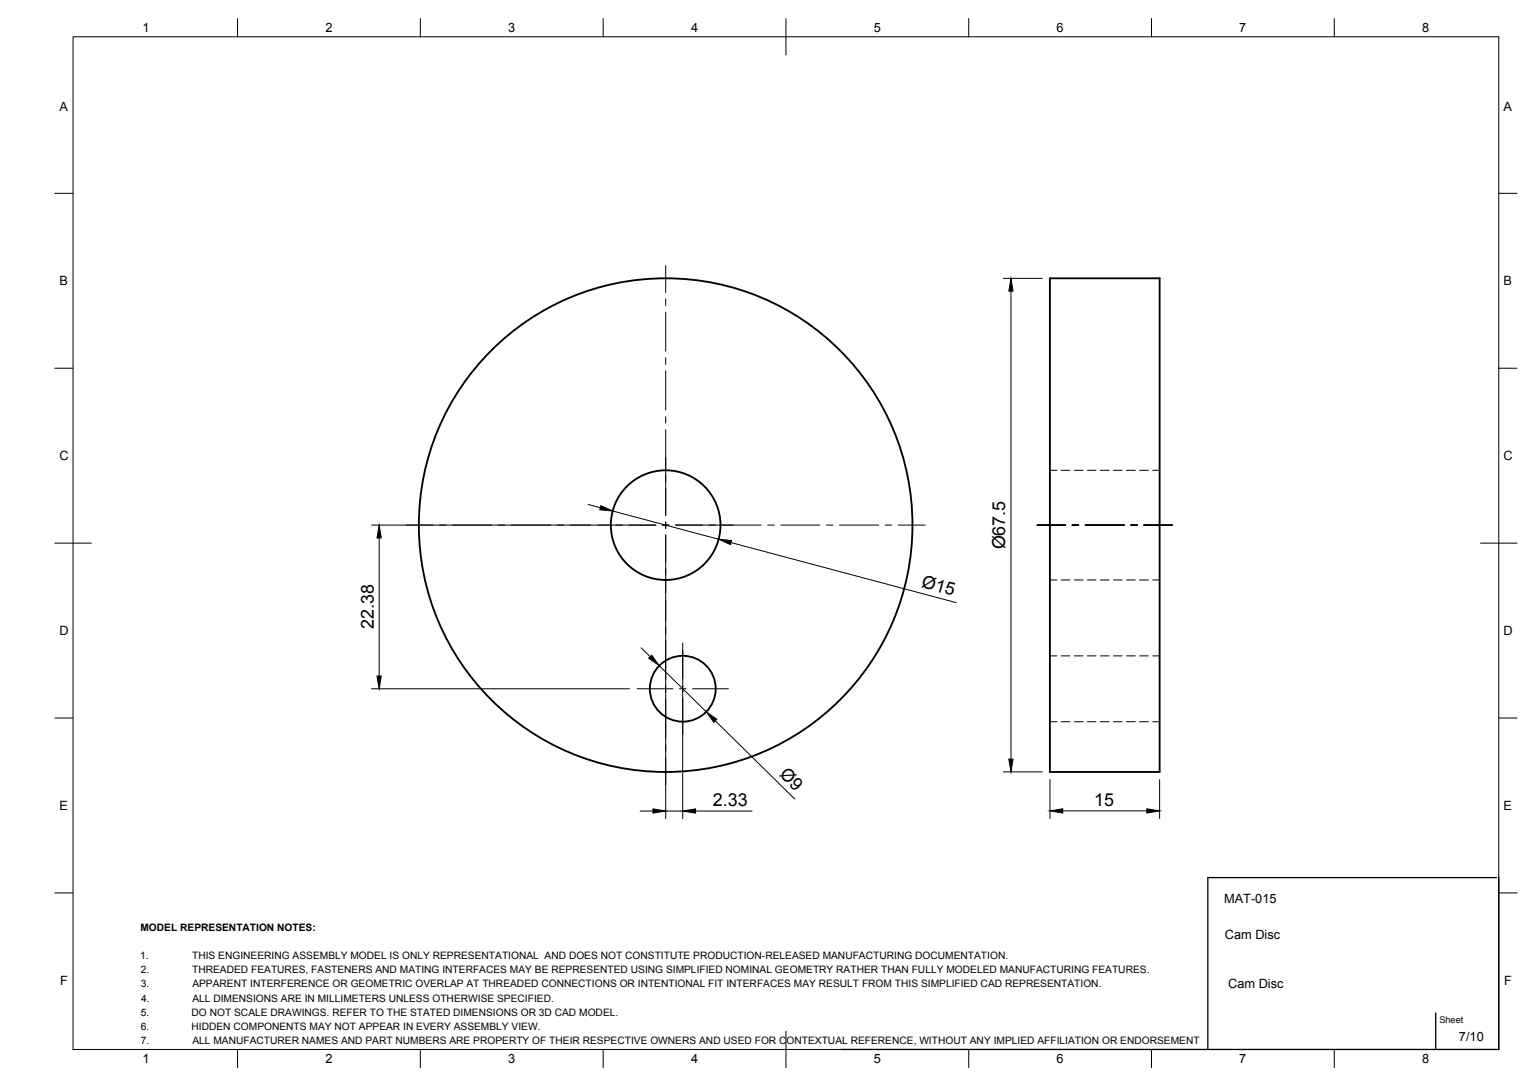
ISO-10303-21;
HEADER;
/* Generated by software containing ST-Developer
 * from STEP Tools, Inc. (www.steptools.com) 
 */

FILE_DESCRIPTION(
/* description */ ('STEP AP214'),
/* implementation_level */ '2;1');

FILE_NAME(
/* name */ 'Cam Disc.step',
/* time_stamp */ '2026-11-14T06:03:18-08:00',
/* author */ (''),
/* organization */ (''),
/* preprocessor_version */ 'ST-DEVELOPER v20.2',
/* originating_system */ 'Autodesk Translation Framework v15.17.0.0',
/* authorisation */ '');

FILE_SCHEMA (('AUTOMOTIVE_DESIGN { 1 0 10303 214 3 1 1 }'));
ENDSEC;

DATA;
#10=MECHANICAL_DESIGN_GEOMETRIC_PRESENTATION_REPRESENTATION('',(#75),#3206);
#59=SHAPE_REPRESENTATION_RELATIONSHIP('SRR','None',#3242,#67);
#67=ADVANCED_BREP_SHAPE_REPRESENTATION('',(#83),#3201);
#75=STYLED_ITEM('',(#3289),#83);
#83=MANIFOLD_SOLID_BREP('Body1',#1782);
#109=PLANE('',#1959);
#110=PLANE('',#1960);
#160=FACE_BOUND('',#666,.T.);
#161=FACE_BOUND('',#667,.T.);
#162=FACE_BOUND('',#669,.T.);
#163=FACE_BOUND('',#670,.T.);
#224=LINE('',#2852,#369);
#225=LINE('',#2858,#370);
#226=LINE('',#2864,#371);
#369=VECTOR('',#2263,4.50000000000001);
#370=VECTOR('',#2270,7.50000000000002);
#371=VECTOR('',#2277,33.7500000000001);
#489=CYLINDRICAL_SURFACE('',#1950,4.50000000000001);
#490=CYLINDRICAL_SURFACE('',#1953,7.50000000000002);
#491=CYLINDRICAL_SURFACE('',#1956,33.7500000000001);
#549=FACE_OUTER_BOUND('',#662,.T.);
#550=FACE_OUTER_BOUND('',#663,.T.);
#551=FACE_OUTER_BOUND('',#664,.T.);
#552=FACE_OUTER_BOUND('',#665,.T.);
#553=FACE_OUTER_BOUND('',#668,.T.);
#662=EDGE_LOOP('',(#1361,#1362,#1363,#1364));
#663=EDGE_LOOP('',(#1365,#1366,#1367,#1368));
#664=EDGE_LOOP('',(#1369,#1370,#1371,#1372));
#665=EDGE_LOOP('',(#1373));
#666=EDGE_LOOP('',(#1374));
#667=EDGE_LOOP('',(#1375));
#668=EDGE_LOOP('',(#1376));
#669=EDGE_LOOP('',(#1377));
#670=EDGE_LOOP('',(#1378));
#785=CIRCLE('',#1951,4.50000000000001);
#786=CIRCLE('',#1952,4.50000000000001);
#787=CIRCLE('',#1954,7.50000000000002);
#788=CIRCLE('',#1955,7.50000000000002);
#789=CIRCLE('',#1957,33.7500000000001);
#790=CIRCLE('',#1958,33.7500000000001);
#882=VERTEX_POINT('',#2849);
#883=VERTEX_POINT('',#2851);
#884=VERTEX_POINT('',#2855);
#885=VERTEX_POINT('',#2857);
#886=VERTEX_POINT('',#2861);
#887=VERTEX_POINT('',#2863);
#1059=EDGE_CURVE('',#882,#882,#785,.T.);
#1060=EDGE_CURVE('',#882,#883,#224,.T.);
#1061=EDGE_CURVE('',#883,#883,#786,.T.);
#1062=EDGE_CURVE('',#884,#884,#787,.T.);
#1063=EDGE_CURVE('',#884,#885,#225,.T.);
#1064=EDGE_CURVE('',#885,#885,#788,.T.);
#1065=EDGE_CURVE('',#886,#886,#789,.T.);
#1066=EDGE_CURVE('',#886,#887,#226,.T.);
#1067=EDGE_CURVE('',#887,#887,#790,.T.);
#1361=ORIENTED_EDGE('',*,*,#1059,.T.);
#1362=ORIENTED_EDGE('',*,*,#1060,.T.);
#1363=ORIENTED_EDGE('',*,*,#1061,.F.);
#1364=ORIENTED_EDGE('',*,*,#1060,.F.);
#1365=ORIENTED_EDGE('',*,*,#1062,.T.);
#1366=ORIENTED_EDGE('',*,*,#1063,.T.);
#1367=ORIENTED_EDGE('',*,*,#1064,.F.);
#1368=ORIENTED_EDGE('',*,*,#1063,.F.);
#1369=ORIENTED_EDGE('',*,*,#1065,.T.);
#1370=ORIENTED_EDGE('',*,*,#1066,.T.);
#1371=ORIENTED_EDGE('',*,*,#1067,.F.);
#1372=ORIENTED_EDGE('',*,*,#1066,.F.);
#1373=ORIENTED_EDGE('',*,*,#1067,.T.);
#1374=ORIENTED_EDGE('',*,*,#1059,.F.);
#1375=ORIENTED_EDGE('',*,*,#1062,.F.);
#1376=ORIENTED_EDGE('',*,*,#1065,.F.);
#1377=ORIENTED_EDGE('',*,*,#1061,.T.);
#1378=ORIENTED_EDGE('',*,*,#1064,.T.);
#1716=ADVANCED_FACE('',(#549),#489,.F.);
#1717=ADVANCED_FACE('',(#550),#490,.F.);
#1718=ADVANCED_FACE('',(#551),#491,.T.);
#1719=ADVANCED_FACE('',(#552,#160,#161),#109,.T.);
#1720=ADVANCED_FACE('',(#553,#162,#163),#110,.F.);
#1782=CLOSED_SHELL('',(#1716,#1717,#1718,#1719,#1720));
#1949=AXIS2_PLACEMENT_3D('',#2847,#2257,#2258);
#1950=AXIS2_PLACEMENT_3D('',#2848,#2259,#2260);
#1951=AXIS2_PLACEMENT_3D('',#2850,#2261,#2262);
#1952=AXIS2_PLACEMENT_3D('',#2853,#2264,#2265);
#1953=AXIS2_PLACEMENT_3D('',#2854,#2266,#2267);
#1954=AXIS2_PLACEMENT_3D('',#2856,#2268,#2269);
#1955=AXIS2_PLACEMENT_3D('',#2859,#2271,#2272);
#1956=AXIS2_PLACEMENT_3D('',#2860,#2273,#2274);
#1957=AXIS2_PLACEMENT_3D('',#2862,#2275,#2276);
#1958=AXIS2_PLACEMENT_3D('',#2865,#2278,#2279);
#1959=AXIS2_PLACEMENT_3D('',#2866,#2280,#2281);
#1960=AXIS2_PLACEMENT_3D('',#2867,#2282,#2283);
#2257=DIRECTION('axis',(0.,0.,1.));
#2258=DIRECTION('refdir',(1.,0.,0.));
#2259=DIRECTION('center_axis',(-1.87200390594439E-31,-2.8065614114583E-31,
-1.));
#2260=DIRECTION('ref_axis',(-1.,5.25389392452275E-62,1.87200390594439E-31));
#2261=DIRECTION('center_axis',(1.87200390594439E-31,2.8065614114583E-31,
1.));
#2262=DIRECTION('ref_axis',(1.,-5.25389392452275E-62,-1.87200390594439E-31));
#2263=DIRECTION('',(-1.87200390594439E-31,-2.8065614114583E-31,-1.));
#2264=DIRECTION('center_axis',(1.87200390594439E-31,2.8065614114583E-31,
1.));
#2265=DIRECTION('ref_axis',(1.,-5.25389392452275E-62,-1.87200390594439E-31));
#2266=DIRECTION('center_axis',(-1.87200390594439E-31,-2.8065614114583E-31,
-1.));
#2267=DIRECTION('ref_axis',(-1.,-2.89120579329467E-17,1.87200390594439E-31));
#2268=DIRECTION('center_axis',(1.87200390594439E-31,2.8065614114583E-31,
1.));
#2269=DIRECTION('ref_axis',(1.,2.89120579329467E-17,-1.87200390594439E-31));
#2270=DIRECTION('',(-1.87200390594439E-31,-2.8065614114583E-31,-1.));
#2271=DIRECTION('center_axis',(1.87200390594439E-31,2.8065614114583E-31,
1.));
#2272=DIRECTION('ref_axis',(1.,2.89120579329467E-17,-1.87200390594439E-31));
#2273=DIRECTION('center_axis',(-1.87200390594439E-31,-2.8065614114583E-31,
-1.));
#2274=DIRECTION('ref_axis',(-1.,-2.81089452125871E-17,1.87200390594439E-31));
#2275=DIRECTION('center_axis',(1.87200390594439E-31,2.8065614114583E-31,
1.));
#2276=DIRECTION('ref_axis',(1.,2.81089452125871E-17,-1.87200390594439E-31));
#2277=DIRECTION('',(1.87200390594439E-31,2.8065614114583E-31,1.));
#2278=DIRECTION('center_axis',(1.87200390594439E-31,2.8065614114583E-31,
1.));
#2279=DIRECTION('ref_axis',(1.,2.81089452125871E-17,-1.87200390594439E-31));
#2280=DIRECTION('center_axis',(-1.85852239633368E-31,2.8065614114583E-31,
1.));
#2281=DIRECTION('ref_axis',(1.,2.77555756156288E-17,1.85852239633368E-31));
#2282=DIRECTION('center_axis',(-1.85852239633368E-31,2.8065614114583E-31,
1.));
#2283=DIRECTION('ref_axis',(1.,2.77555756156288E-17,1.85852239633368E-31));
#2847=CARTESIAN_POINT('',(0.,0.,0.));
#2848=CARTESIAN_POINT('Origin',(-6.93889390390723E-15,22.6429327686607,
12.5));
#2849=CARTESIAN_POINT('',(4.50000000000001,22.6429327686607,12.5));
#2850=CARTESIAN_POINT('Origin',(-6.93889390390723E-15,22.6429327686607,
12.5));
#2851=CARTESIAN_POINT('',(4.50000000000001,22.6429327686607,-2.5));
#2852=CARTESIAN_POINT('',(4.50000000000001,22.6429327686607,12.5));
#2853=CARTESIAN_POINT('Origin',(-6.93889390390723E-15,22.6429327686607,
-2.5));
#2854=CARTESIAN_POINT('Origin',(0.,0.142932768660666,12.5));
#2855=CARTESIAN_POINT('',(7.50000000000002,0.142932768660665,12.5));
#2856=CARTESIAN_POINT('Origin',(0.,0.142932768660666,12.5));
#2857=CARTESIAN_POINT('',(7.50000000000002,0.142932768660665,-2.5));
#2858=CARTESIAN_POINT('',(7.50000000000002,0.142932768660665,12.5));
#2859=CARTESIAN_POINT('Origin',(0.,0.142932768660666,-2.5));
#2860=CARTESIAN_POINT('Origin',(0.,0.142932768660666,12.5));
#2861=CARTESIAN_POINT('',(33.7500000000001,0.142932768660662,-2.5));
#2862=CARTESIAN_POINT('Origin',(0.,0.142932768660666,-2.5));
#2863=CARTESIAN_POINT('',(33.7500000000001,0.142932768660662,12.5));
#2864=CARTESIAN_POINT('',(33.7500000000001,0.142932768660662,12.5));
#2865=CARTESIAN_POINT('Origin',(0.,0.142932768660666,12.5));
#2866=CARTESIAN_POINT('Origin',(0.,0.142932768660666,12.5));
#2867=CARTESIAN_POINT('Origin',(0.,0.142932768660666,-2.5));
#3191=UNCERTAINTY_MEASURE_WITH_UNIT(LENGTH_MEASURE(0.01),#3207,
'DISTANCE_ACCURACY_VALUE',
'Maximum model space distance between geometric entities at asserted c
onnectivities');
#3196=UNCERTAINTY_MEASURE_WITH_UNIT(LENGTH_MEASURE(0.01),#3207,
'DISTANCE_ACCURACY_VALUE',
'Maximum model space distance between geometric entities at asserted c
onnectivities');
#3201=(
GEOMETRIC_REPRESENTATION_CONTEXT(3)
GLOBAL_UNCERTAINTY_ASSIGNED_CONTEXT((#3191))
GLOBAL_UNIT_ASSIGNED_CONTEXT((#3207,#3209,#3210))
REPRESENTATION_CONTEXT('','3D')
);
#3206=(
GEOMETRIC_REPRESENTATION_CONTEXT(3)
GLOBAL_UNCERTAINTY_ASSIGNED_CONTEXT((#3196))
GLOBAL_UNIT_ASSIGNED_CONTEXT((#3207,#3209,#3210))
REPRESENTATION_CONTEXT('','3D')
);
#3207=(
LENGTH_UNIT()
NAMED_UNIT(*)
SI_UNIT(.MILLI.,.METRE.)
);
#3209=(
NAMED_UNIT(*)
PLANE_ANGLE_UNIT()
SI_UNIT($,.RADIAN.)
);
#3210=(
NAMED_UNIT(*)
SI_UNIT($,.STERADIAN.)
SOLID_ANGLE_UNIT()
);
#3215=SHAPE_DEFINITION_REPRESENTATION(#3224,#3242);
#3224=PRODUCT_DEFINITION_SHAPE('',$,#3252);
#3242=SHAPE_REPRESENTATION('',(#1949),#3201);
#3247=PRODUCT_DEFINITION_CONTEXT('part definition',#3276,'design');
#3252=PRODUCT_DEFINITION('Cam Disc','Cam Disc',#3261,#3247);
#3261=PRODUCT_DEFINITION_FORMATION('',$,#3282);
#3276=APPLICATION_CONTEXT(
'Core Data for Automotive Mechanical Design Process');
#3277=PRODUCT_CONTEXT('part definition',#3276,'mechanical');
#3282=PRODUCT('Cam Disc','Cam Disc',$,(#3277));
#3289=PRESENTATION_STYLE_ASSIGNMENT((#3293));
#3293=SURFACE_STYLE_USAGE(.BOTH.,#3297);
#3297=SURFACE_SIDE_STYLE('',(#3301));
#3301=SURFACE_STYLE_FILL_AREA(#3305);
#3305=FILL_AREA_STYLE('Opaque(97,158,199)',(#3309));
#3309=FILL_AREA_STYLE_COLOUR('Opaque(97,158,199)',#3313);
#3313=COLOUR_RGB('Opaque(97,158,199)',0.380392156862745,0.619607843137255,
0.780392156862745);
ENDSEC;
END-ISO-10303-21;
